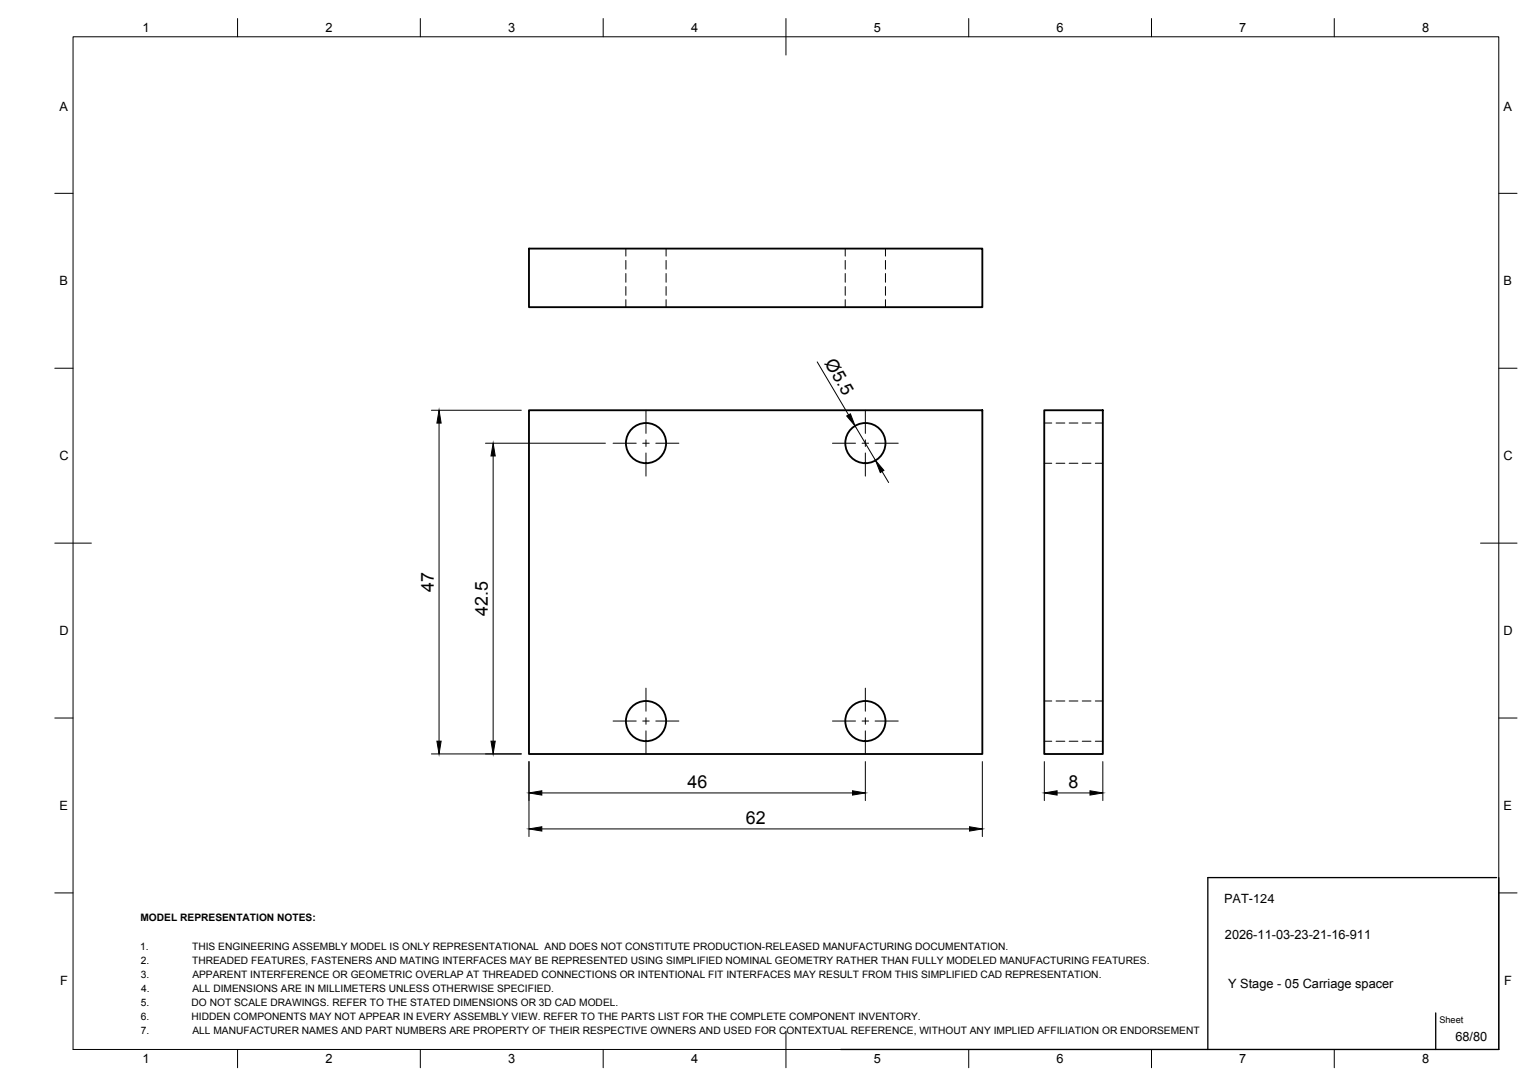
ISO-10303-21;
HEADER;
/* Generated by software containing ST-Developer
 * from STEP Tools, Inc. (www.steptools.com) 
 */

FILE_DESCRIPTION(
/* description */ ('XY cross-slide table'),
/* implementation_level */ '2;1');

FILE_NAME(
/* name */ 'Y Stage - 05 Carriage spacer.step',
/* time_stamp */ '2026-10-28T03:22:46-07:00',
/* author */ (''),
/* organization */ (''),
/* preprocessor_version */ 'ST-DEVELOPER v20.2',
/* originating_system */ 'Autodesk Translation Framework v15.17.0.0',
/* authorisation */ '');

FILE_SCHEMA (('AUTOMOTIVE_DESIGN { 1 0 10303 214 3 1 1 }'));
ENDSEC;

DATA;
#10=MECHANICAL_DESIGN_GEOMETRIC_PRESENTATION_REPRESENTATION('',(#1762),#62984);
#1566=SHAPE_REPRESENTATION_RELATIONSHIP('SRR','None',#63424,#1649);
#1649=ADVANCED_BREP_SHAPE_REPRESENTATION('',(#1870),#62961);
#1762=STYLED_ITEM('',(#63898),#1870);
#1870=MANIFOLD_SOLID_BREP('Body1',#23061);
#2220=FACE_BOUND('',#5446,.T.);
#2221=FACE_BOUND('',#5447,.T.);
#2222=FACE_BOUND('',#5448,.T.);
#2223=FACE_BOUND('',#5449,.T.);
#2224=FACE_BOUND('',#5451,.T.);
#2225=FACE_BOUND('',#5452,.T.);
#2226=FACE_BOUND('',#5453,.T.);
#2227=FACE_BOUND('',#5454,.T.);
#2706=PLANE('',#25830);
#2707=PLANE('',#25831);
#2708=PLANE('',#25832);
#2709=PLANE('',#25833);
#2710=PLANE('',#25834);
#2711=PLANE('',#25835);
#3790=FACE_OUTER_BOUND('',#5437,.T.);
#3791=FACE_OUTER_BOUND('',#5438,.T.);
#3792=FACE_OUTER_BOUND('',#5439,.T.);
#3793=FACE_OUTER_BOUND('',#5440,.T.);
#3794=FACE_OUTER_BOUND('',#5441,.T.);
#3795=FACE_OUTER_BOUND('',#5442,.T.);
#3796=FACE_OUTER_BOUND('',#5443,.T.);
#3797=FACE_OUTER_BOUND('',#5444,.T.);
#3798=FACE_OUTER_BOUND('',#5445,.T.);
#3799=FACE_OUTER_BOUND('',#5450,.T.);
#5437=EDGE_LOOP('',(#19098,#19099,#19100,#19101));
#5438=EDGE_LOOP('',(#19102,#19103,#19104,#19105));
#5439=EDGE_LOOP('',(#19106,#19107,#19108,#19109));
#5440=EDGE_LOOP('',(#19110,#19111,#19112,#19113));
#5441=EDGE_LOOP('',(#19114,#19115,#19116,#19117));
#5442=EDGE_LOOP('',(#19118,#19119,#19120,#19121));
#5443=EDGE_LOOP('',(#19122,#19123,#19124,#19125));
#5444=EDGE_LOOP('',(#19126,#19127,#19128,#19129));
#5445=EDGE_LOOP('',(#19130,#19131,#19132,#19133));
#5446=EDGE_LOOP('',(#19134));
#5447=EDGE_LOOP('',(#19135));
#5448=EDGE_LOOP('',(#19136));
#5449=EDGE_LOOP('',(#19137));
#5450=EDGE_LOOP('',(#19138,#19139,#19140,#19141));
#5451=EDGE_LOOP('',(#19142));
#5452=EDGE_LOOP('',(#19143));
#5453=EDGE_LOOP('',(#19144));
#5454=EDGE_LOOP('',(#19145));
#6892=LINE('',#49716,#8379);
#6893=LINE('',#49722,#8380);
#6894=LINE('',#49728,#8381);
#6895=LINE('',#49734,#8382);
#6896=LINE('',#49739,#8383);
#6897=LINE('',#49741,#8384);
#6898=LINE('',#49743,#8385);
#6899=LINE('',#49744,#8386);
#6900=LINE('',#49747,#8387);
#6901=LINE('',#49749,#8388);
#6902=LINE('',#49750,#8389);
#6903=LINE('',#49753,#8390);
#6904=LINE('',#49755,#8391);
#6905=LINE('',#49756,#8392);
#6906=LINE('',#49758,#8393);
#6907=LINE('',#49759,#8394);
#8379=VECTOR('',#31087,0.275);
#8380=VECTOR('',#31094,0.275);
#8381=VECTOR('',#31101,0.275);
#8382=VECTOR('',#31108,0.275);
#8383=VECTOR('',#31113,1.);
#8384=VECTOR('',#31114,1.);
#8385=VECTOR('',#31115,1.);
#8386=VECTOR('',#31116,1.);
#8387=VECTOR('',#31119,1.);
#8388=VECTOR('',#31120,1.);
#8389=VECTOR('',#31121,1.);
#8390=VECTOR('',#31124,1.);
#8391=VECTOR('',#31125,1.);
#8392=VECTOR('',#31126,1.);
#8393=VECTOR('',#31129,1.);
#8394=VECTOR('',#31130,1.);
#9615=CIRCLE('',#25819,0.275);
#9616=CIRCLE('',#25820,0.275);
#9617=CIRCLE('',#25822,0.275);
#9618=CIRCLE('',#25823,0.275);
#9619=CIRCLE('',#25825,0.275);
#9620=CIRCLE('',#25826,0.275);
#9621=CIRCLE('',#25828,0.275);
#9622=CIRCLE('',#25829,0.275);
#11194=VERTEX_POINT('',#49713);
#11195=VERTEX_POINT('',#49715);
#11196=VERTEX_POINT('',#49719);
#11197=VERTEX_POINT('',#49721);
#11198=VERTEX_POINT('',#49725);
#11199=VERTEX_POINT('',#49727);
#11200=VERTEX_POINT('',#49731);
#11201=VERTEX_POINT('',#49733);
#11202=VERTEX_POINT('',#49737);
#11203=VERTEX_POINT('',#49738);
#11204=VERTEX_POINT('',#49740);
#11205=VERTEX_POINT('',#49742);
#11206=VERTEX_POINT('',#49746);
#11207=VERTEX_POINT('',#49748);
#11208=VERTEX_POINT('',#49752);
#11209=VERTEX_POINT('',#49754);
#13933=EDGE_CURVE('',#11194,#11194,#9615,.T.);
#13934=EDGE_CURVE('',#11194,#11195,#6892,.T.);
#13935=EDGE_CURVE('',#11195,#11195,#9616,.T.);
#13936=EDGE_CURVE('',#11196,#11196,#9617,.T.);
#13937=EDGE_CURVE('',#11196,#11197,#6893,.T.);
#13938=EDGE_CURVE('',#11197,#11197,#9618,.T.);
#13939=EDGE_CURVE('',#11198,#11198,#9619,.T.);
#13940=EDGE_CURVE('',#11198,#11199,#6894,.T.);
#13941=EDGE_CURVE('',#11199,#11199,#9620,.T.);
#13942=EDGE_CURVE('',#11200,#11200,#9621,.T.);
#13943=EDGE_CURVE('',#11200,#11201,#6895,.T.);
#13944=EDGE_CURVE('',#11201,#11201,#9622,.T.);
#13945=EDGE_CURVE('',#11202,#11203,#6896,.T.);
#13946=EDGE_CURVE('',#11203,#11204,#6897,.T.);
#13947=EDGE_CURVE('',#11205,#11204,#6898,.T.);
#13948=EDGE_CURVE('',#11202,#11205,#6899,.T.);
#13949=EDGE_CURVE('',#11206,#11202,#6900,.T.);
#13950=EDGE_CURVE('',#11207,#11205,#6901,.T.);
#13951=EDGE_CURVE('',#11206,#11207,#6902,.T.);
#13952=EDGE_CURVE('',#11208,#11206,#6903,.T.);
#13953=EDGE_CURVE('',#11209,#11207,#6904,.T.);
#13954=EDGE_CURVE('',#11208,#11209,#6905,.T.);
#13955=EDGE_CURVE('',#11203,#11208,#6906,.T.);
#13956=EDGE_CURVE('',#11204,#11209,#6907,.T.);
#19098=ORIENTED_EDGE('',*,*,#13933,.F.);
#19099=ORIENTED_EDGE('',*,*,#13934,.T.);
#19100=ORIENTED_EDGE('',*,*,#13935,.F.);
#19101=ORIENTED_EDGE('',*,*,#13934,.F.);
#19102=ORIENTED_EDGE('',*,*,#13936,.F.);
#19103=ORIENTED_EDGE('',*,*,#13937,.T.);
#19104=ORIENTED_EDGE('',*,*,#13938,.F.);
#19105=ORIENTED_EDGE('',*,*,#13937,.F.);
#19106=ORIENTED_EDGE('',*,*,#13939,.F.);
#19107=ORIENTED_EDGE('',*,*,#13940,.T.);
#19108=ORIENTED_EDGE('',*,*,#13941,.F.);
#19109=ORIENTED_EDGE('',*,*,#13940,.F.);
#19110=ORIENTED_EDGE('',*,*,#13942,.F.);
#19111=ORIENTED_EDGE('',*,*,#13943,.T.);
#19112=ORIENTED_EDGE('',*,*,#13944,.F.);
#19113=ORIENTED_EDGE('',*,*,#13943,.F.);
#19114=ORIENTED_EDGE('',*,*,#13945,.T.);
#19115=ORIENTED_EDGE('',*,*,#13946,.T.);
#19116=ORIENTED_EDGE('',*,*,#13947,.F.);
#19117=ORIENTED_EDGE('',*,*,#13948,.F.);
#19118=ORIENTED_EDGE('',*,*,#13949,.T.);
#19119=ORIENTED_EDGE('',*,*,#13948,.T.);
#19120=ORIENTED_EDGE('',*,*,#13950,.F.);
#19121=ORIENTED_EDGE('',*,*,#13951,.F.);
#19122=ORIENTED_EDGE('',*,*,#13952,.T.);
#19123=ORIENTED_EDGE('',*,*,#13951,.T.);
#19124=ORIENTED_EDGE('',*,*,#13953,.F.);
#19125=ORIENTED_EDGE('',*,*,#13954,.F.);
#19126=ORIENTED_EDGE('',*,*,#13955,.T.);
#19127=ORIENTED_EDGE('',*,*,#13954,.T.);
#19128=ORIENTED_EDGE('',*,*,#13956,.F.);
#19129=ORIENTED_EDGE('',*,*,#13946,.F.);
#19130=ORIENTED_EDGE('',*,*,#13956,.T.);
#19131=ORIENTED_EDGE('',*,*,#13953,.T.);
#19132=ORIENTED_EDGE('',*,*,#13950,.T.);
#19133=ORIENTED_EDGE('',*,*,#13947,.T.);
#19134=ORIENTED_EDGE('',*,*,#13935,.T.);
#19135=ORIENTED_EDGE('',*,*,#13938,.T.);
#19136=ORIENTED_EDGE('',*,*,#13941,.T.);
#19137=ORIENTED_EDGE('',*,*,#13944,.T.);
#19138=ORIENTED_EDGE('',*,*,#13955,.F.);
#19139=ORIENTED_EDGE('',*,*,#13945,.F.);
#19140=ORIENTED_EDGE('',*,*,#13949,.F.);
#19141=ORIENTED_EDGE('',*,*,#13952,.F.);
#19142=ORIENTED_EDGE('',*,*,#13933,.T.);
#19143=ORIENTED_EDGE('',*,*,#13936,.T.);
#19144=ORIENTED_EDGE('',*,*,#13939,.T.);
#19145=ORIENTED_EDGE('',*,*,#13942,.T.);
#21442=CYLINDRICAL_SURFACE('',#25818,0.275);
#21443=CYLINDRICAL_SURFACE('',#25821,0.275);
#21444=CYLINDRICAL_SURFACE('',#25824,0.275);
#21445=CYLINDRICAL_SURFACE('',#25827,0.275);
#22571=ADVANCED_FACE('',(#3790),#21442,.F.);
#22572=ADVANCED_FACE('',(#3791),#21443,.F.);
#22573=ADVANCED_FACE('',(#3792),#21444,.F.);
#22574=ADVANCED_FACE('',(#3793),#21445,.F.);
#22575=ADVANCED_FACE('',(#3794),#2706,.T.);
#22576=ADVANCED_FACE('',(#3795),#2707,.T.);
#22577=ADVANCED_FACE('',(#3796),#2708,.T.);
#22578=ADVANCED_FACE('',(#3797),#2709,.T.);
#22579=ADVANCED_FACE('',(#3798,#2220,#2221,#2222,#2223),#2710,.T.);
#22580=ADVANCED_FACE('',(#3799,#2224,#2225,#2226,#2227),#2711,.F.);
#23061=CLOSED_SHELL('',(#22571,#22572,#22573,#22574,#22575,#22576,#22577,
#22578,#22579,#22580));
#25817=AXIS2_PLACEMENT_3D('',#49711,#31081,#31082);
#25818=AXIS2_PLACEMENT_3D('',#49712,#31083,#31084);
#25819=AXIS2_PLACEMENT_3D('',#49714,#31085,#31086);
#25820=AXIS2_PLACEMENT_3D('',#49717,#31088,#31089);
#25821=AXIS2_PLACEMENT_3D('',#49718,#31090,#31091);
#25822=AXIS2_PLACEMENT_3D('',#49720,#31092,#31093);
#25823=AXIS2_PLACEMENT_3D('',#49723,#31095,#31096);
#25824=AXIS2_PLACEMENT_3D('',#49724,#31097,#31098);
#25825=AXIS2_PLACEMENT_3D('',#49726,#31099,#31100);
#25826=AXIS2_PLACEMENT_3D('',#49729,#31102,#31103);
#25827=AXIS2_PLACEMENT_3D('',#49730,#31104,#31105);
#25828=AXIS2_PLACEMENT_3D('',#49732,#31106,#31107);
#25829=AXIS2_PLACEMENT_3D('',#49735,#31109,#31110);
#25830=AXIS2_PLACEMENT_3D('',#49736,#31111,#31112);
#25831=AXIS2_PLACEMENT_3D('',#49745,#31117,#31118);
#25832=AXIS2_PLACEMENT_3D('',#49751,#31122,#31123);
#25833=AXIS2_PLACEMENT_3D('',#49757,#31127,#31128);
#25834=AXIS2_PLACEMENT_3D('',#49760,#31131,#31132);
#25835=AXIS2_PLACEMENT_3D('',#49761,#31133,#31134);
#31081=DIRECTION('axis',(0.,0.,1.));
#31082=DIRECTION('refdir',(1.,0.,0.));
#31083=DIRECTION('center_axis',(0.,0.,1.));
#31084=DIRECTION('ref_axis',(1.,0.,0.));
#31085=DIRECTION('center_axis',(0.,0.,1.));
#31086=DIRECTION('ref_axis',(1.,0.,0.));
#31087=DIRECTION('',(0.,0.,1.));
#31088=DIRECTION('center_axis',(0.,0.,-1.));
#31089=DIRECTION('ref_axis',(1.,0.,0.));
#31090=DIRECTION('center_axis',(0.,0.,1.));
#31091=DIRECTION('ref_axis',(1.,0.,0.));
#31092=DIRECTION('center_axis',(0.,0.,1.));
#31093=DIRECTION('ref_axis',(1.,0.,0.));
#31094=DIRECTION('',(0.,0.,1.));
#31095=DIRECTION('center_axis',(0.,0.,-1.));
#31096=DIRECTION('ref_axis',(1.,0.,0.));
#31097=DIRECTION('center_axis',(0.,0.,1.));
#31098=DIRECTION('ref_axis',(1.,0.,0.));
#31099=DIRECTION('center_axis',(0.,0.,1.));
#31100=DIRECTION('ref_axis',(1.,0.,0.));
#31101=DIRECTION('',(0.,0.,1.));
#31102=DIRECTION('center_axis',(0.,0.,-1.));
#31103=DIRECTION('ref_axis',(1.,0.,0.));
#31104=DIRECTION('center_axis',(0.,0.,1.));
#31105=DIRECTION('ref_axis',(1.,0.,0.));
#31106=DIRECTION('center_axis',(0.,0.,1.));
#31107=DIRECTION('ref_axis',(1.,0.,0.));
#31108=DIRECTION('',(0.,0.,1.));
#31109=DIRECTION('center_axis',(0.,0.,-1.));
#31110=DIRECTION('ref_axis',(1.,0.,0.));
#31111=DIRECTION('center_axis',(0.,1.,0.));
#31112=DIRECTION('ref_axis',(-1.,0.,0.));
#31113=DIRECTION('',(-1.,0.,0.));
#31114=DIRECTION('',(0.,0.,1.));
#31115=DIRECTION('',(-1.,0.,0.));
#31116=DIRECTION('',(0.,0.,1.));
#31117=DIRECTION('center_axis',(1.,0.,0.));
#31118=DIRECTION('ref_axis',(0.,1.,0.));
#31119=DIRECTION('',(0.,1.,0.));
#31120=DIRECTION('',(0.,1.,0.));
#31121=DIRECTION('',(0.,0.,1.));
#31122=DIRECTION('center_axis',(0.,-1.,0.));
#31123=DIRECTION('ref_axis',(1.,0.,0.));
#31124=DIRECTION('',(1.,0.,0.));
#31125=DIRECTION('',(1.,0.,0.));
#31126=DIRECTION('',(0.,0.,1.));
#31127=DIRECTION('center_axis',(-1.,0.,0.));
#31128=DIRECTION('ref_axis',(0.,-1.,0.));
#31129=DIRECTION('',(0.,-1.,0.));
#31130=DIRECTION('',(0.,-1.,0.));
#31131=DIRECTION('center_axis',(0.,0.,1.));
#31132=DIRECTION('ref_axis',(1.,0.,0.));
#31133=DIRECTION('center_axis',(0.,0.,1.));
#31134=DIRECTION('ref_axis',(1.,0.,0.));
#49711=CARTESIAN_POINT('',(0.,0.,0.));
#49712=CARTESIAN_POINT('Origin',(15.,-7.9,5.1));
#49713=CARTESIAN_POINT('',(14.725,-7.9,5.2));
#49714=CARTESIAN_POINT('Origin',(15.,-7.9,5.2));
#49715=CARTESIAN_POINT('',(14.725,-7.9,6.));
#49716=CARTESIAN_POINT('',(14.725,-7.9,5.1));
#49717=CARTESIAN_POINT('Origin',(15.,-7.9,6.));
#49718=CARTESIAN_POINT('Origin',(12.,-4.1,5.1));
#49719=CARTESIAN_POINT('',(11.725,-4.1,5.2));
#49720=CARTESIAN_POINT('Origin',(12.,-4.1,5.2));
#49721=CARTESIAN_POINT('',(11.725,-4.1,6.));
#49722=CARTESIAN_POINT('',(11.725,-4.1,5.1));
#49723=CARTESIAN_POINT('Origin',(12.,-4.1,6.));
#49724=CARTESIAN_POINT('Origin',(12.,-7.9,5.1));
#49725=CARTESIAN_POINT('',(11.725,-7.9,5.2));
#49726=CARTESIAN_POINT('Origin',(12.,-7.9,5.2));
#49727=CARTESIAN_POINT('',(11.725,-7.9,6.));
#49728=CARTESIAN_POINT('',(11.725,-7.9,5.1));
#49729=CARTESIAN_POINT('Origin',(12.,-7.9,6.));
#49730=CARTESIAN_POINT('Origin',(15.,-4.1,5.1));
#49731=CARTESIAN_POINT('',(14.725,-4.1,5.2));
#49732=CARTESIAN_POINT('Origin',(15.,-4.1,5.2));
#49733=CARTESIAN_POINT('',(14.725,-4.1,6.));
#49734=CARTESIAN_POINT('',(14.725,-4.1,5.1));
#49735=CARTESIAN_POINT('Origin',(15.,-4.1,6.));
#49736=CARTESIAN_POINT('Origin',(16.6,-3.65,5.2));
#49737=CARTESIAN_POINT('',(16.6,-3.65,5.2));
#49738=CARTESIAN_POINT('',(10.4,-3.65,5.2));
#49739=CARTESIAN_POINT('',(16.6,-3.65,5.2));
#49740=CARTESIAN_POINT('',(10.4,-3.65,6.));
#49741=CARTESIAN_POINT('',(10.4,-3.65,5.2));
#49742=CARTESIAN_POINT('',(16.6,-3.65,6.));
#49743=CARTESIAN_POINT('',(16.6,-3.65,6.));
#49744=CARTESIAN_POINT('',(16.6,-3.65,5.2));
#49745=CARTESIAN_POINT('Origin',(16.6,-8.35,5.2));
#49746=CARTESIAN_POINT('',(16.6,-8.35,5.2));
#49747=CARTESIAN_POINT('',(16.6,-8.35,5.2));
#49748=CARTESIAN_POINT('',(16.6,-8.35,6.));
#49749=CARTESIAN_POINT('',(16.6,-8.35,6.));
#49750=CARTESIAN_POINT('',(16.6,-8.35,5.2));
#49751=CARTESIAN_POINT('Origin',(10.4,-8.35,5.2));
#49752=CARTESIAN_POINT('',(10.4,-8.35,5.2));
#49753=CARTESIAN_POINT('',(10.4,-8.35,5.2));
#49754=CARTESIAN_POINT('',(10.4,-8.35,6.));
#49755=CARTESIAN_POINT('',(10.4,-8.35,6.));
#49756=CARTESIAN_POINT('',(10.4,-8.35,5.2));
#49757=CARTESIAN_POINT('Origin',(10.4,-3.65,5.2));
#49758=CARTESIAN_POINT('',(10.4,-3.65,5.2));
#49759=CARTESIAN_POINT('',(10.4,-3.65,6.));
#49760=CARTESIAN_POINT('Origin',(13.5,-6.,6.));
#49761=CARTESIAN_POINT('Origin',(13.5,-6.,5.2));
#62862=UNCERTAINTY_MEASURE_WITH_UNIT(LENGTH_MEASURE(0.001),#62985,
'DISTANCE_ACCURACY_VALUE',
'Maximum model space distance between geometric entities at asserted c
onnectivities');
#62885=UNCERTAINTY_MEASURE_WITH_UNIT(LENGTH_MEASURE(0.001),#62985,
'DISTANCE_ACCURACY_VALUE',
'Maximum model space distance between geometric entities at asserted c
onnectivities');
#62961=(
GEOMETRIC_REPRESENTATION_CONTEXT(3)
GLOBAL_UNCERTAINTY_ASSIGNED_CONTEXT((#62862))
GLOBAL_UNIT_ASSIGNED_CONTEXT((#62985,#62987,#62988))
REPRESENTATION_CONTEXT('','3D')
);
#62984=(
GEOMETRIC_REPRESENTATION_CONTEXT(3)
GLOBAL_UNCERTAINTY_ASSIGNED_CONTEXT((#62885))
GLOBAL_UNIT_ASSIGNED_CONTEXT((#62985,#62987,#62988))
REPRESENTATION_CONTEXT('','3D')
);
#62985=(
LENGTH_UNIT()
NAMED_UNIT(*)
SI_UNIT(.CENTI.,.METRE.)
);
#62987=(
NAMED_UNIT(*)
PLANE_ANGLE_UNIT()
SI_UNIT($,.RADIAN.)
);
#62988=(
NAMED_UNIT(*)
SI_UNIT($,.STERADIAN.)
SOLID_ANGLE_UNIT()
);
#63064=SHAPE_DEFINITION_REPRESENTATION(#63252,#63424);
#63252=PRODUCT_DEFINITION_SHAPE('',$,#63523);
#63424=SHAPE_REPRESENTATION('',(#25817),#62961);
#63447=PRODUCT_DEFINITION_CONTEXT('part definition',#63743,'design');
#63523=PRODUCT_DEFINITION('Y Stage - 05 Carriage spacer',
'Y Stage - 05 Carriage spacer',#63621,#63447);
#63621=PRODUCT_DEFINITION_FORMATION('',$,#63820);
#63743=APPLICATION_CONTEXT(
'Core Data for Automotive Mechanical Design Process');
#63744=PRODUCT_CONTEXT('part definition',#63743,'mechanical');
#63820=PRODUCT('Y Stage - 05 Carriage spacer',
'Y Stage - 05 Carriage spacer','Y Stage - 05 Carriage spacer',(#63744));
#63892=COLOUR_RGB('Light Blue',0.38,0.62,0.78);
#63893=FILL_AREA_STYLE_COLOUR('',#63892);
#63894=FILL_AREA_STYLE('',(#63893));
#63895=SURFACE_STYLE_FILL_AREA(#63894);
#63896=SURFACE_SIDE_STYLE('',(#63895));
#63897=SURFACE_STYLE_USAGE(.BOTH.,#63896);
#63898=PRESENTATION_STYLE_ASSIGNMENT((#63897));
ENDSEC;
END-ISO-10303-21;
